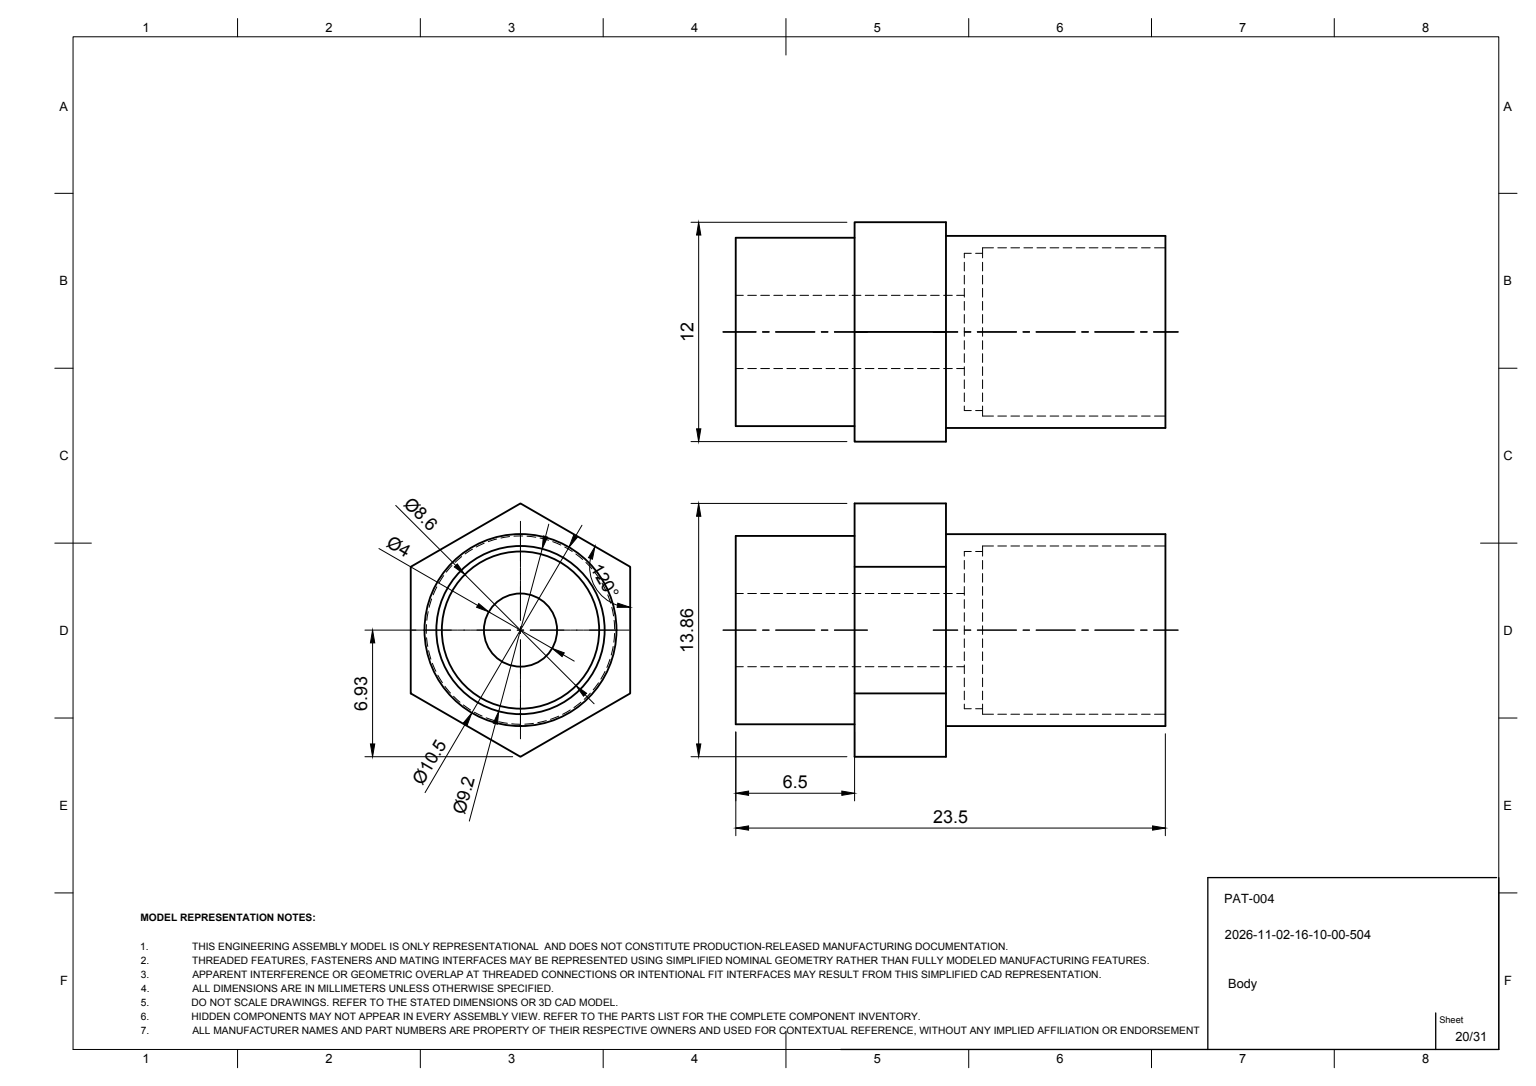
ISO-10303-21;
HEADER;
/* Generated by software containing ST-Developer
 * from STEP Tools, Inc. (www.steptools.com) 
 */

FILE_DESCRIPTION(
/* description */ ('Air blow-off nozzle station'),
/* implementation_level */ '2;1');

FILE_NAME(
/* name */ 'Body.step',
/* time_stamp */ '2026-10-27T10:53:54-07:00',
/* author */ (''),
/* organization */ (''),
/* preprocessor_version */ 'ST-DEVELOPER v20.2',
/* originating_system */ 'Autodesk Translation Framework v15.17.0.0',
/* authorisation */ '');

FILE_SCHEMA (('AUTOMOTIVE_DESIGN { 1 0 10303 214 3 1 1 }'));
ENDSEC;

DATA;
#10=MECHANICAL_DESIGN_GEOMETRIC_PRESENTATION_REPRESENTATION('',(#260),#7897);
#210=SHAPE_REPRESENTATION_RELATIONSHIP('SRR','None',#8028,#235);
#235=ADVANCED_BREP_SHAPE_REPRESENTATION('',(#283),#7895);
#260=STYLED_ITEM('',(#8199),#283);
#283=MANIFOLD_SOLID_BREP('Body1',#4311);
#362=FACE_BOUND('',#1108,.T.);
#363=FACE_BOUND('',#1110,.T.);
#364=FACE_BOUND('',#1112,.T.);
#365=FACE_BOUND('',#1120,.T.);
#366=FACE_BOUND('',#1123,.T.);
#367=FACE_BOUND('',#1127,.T.);
#525=PLANE('',#5017);
#526=PLANE('',#5019);
#527=PLANE('',#5021);
#528=PLANE('',#5023);
#529=PLANE('',#5024);
#530=PLANE('',#5025);
#531=PLANE('',#5026);
#532=PLANE('',#5027);
#533=PLANE('',#5028);
#534=PLANE('',#5029);
#535=PLANE('',#5033);
#536=PLANE('',#5038);
#773=FACE_OUTER_BOUND('',#1106,.T.);
#774=FACE_OUTER_BOUND('',#1107,.T.);
#775=FACE_OUTER_BOUND('',#1109,.T.);
#776=FACE_OUTER_BOUND('',#1111,.T.);
#777=FACE_OUTER_BOUND('',#1113,.T.);
#778=FACE_OUTER_BOUND('',#1114,.T.);
#779=FACE_OUTER_BOUND('',#1115,.T.);
#780=FACE_OUTER_BOUND('',#1116,.T.);
#781=FACE_OUTER_BOUND('',#1117,.T.);
#782=FACE_OUTER_BOUND('',#1118,.T.);
#783=FACE_OUTER_BOUND('',#1119,.T.);
#784=FACE_OUTER_BOUND('',#1121,.T.);
#785=FACE_OUTER_BOUND('',#1122,.T.);
#786=FACE_OUTER_BOUND('',#1124,.T.);
#787=FACE_OUTER_BOUND('',#1125,.T.);
#788=FACE_OUTER_BOUND('',#1126,.T.);
#789=FACE_OUTER_BOUND('',#1128,.T.);
#1106=EDGE_LOOP('',(#3875,#3876,#3877,#3878));
#1107=EDGE_LOOP('',(#3879));
#1108=EDGE_LOOP('',(#3880));
#1109=EDGE_LOOP('',(#3881,#3882,#3883,#3884,#3885,#3886));
#1110=EDGE_LOOP('',(#3887));
#1111=EDGE_LOOP('',(#3888,#3889,#3890,#3891,#3892,#3893));
#1112=EDGE_LOOP('',(#3894));
#1113=EDGE_LOOP('',(#3895,#3896,#3897,#3898));
#1114=EDGE_LOOP('',(#3899,#3900,#3901,#3902));
#1115=EDGE_LOOP('',(#3903,#3904,#3905,#3906));
#1116=EDGE_LOOP('',(#3907,#3908,#3909,#3910));
#1117=EDGE_LOOP('',(#3911,#3912,#3913,#3914));
#1118=EDGE_LOOP('',(#3915,#3916,#3917,#3918));
#1119=EDGE_LOOP('',(#3919));
#1120=EDGE_LOOP('',(#3920));
#1121=EDGE_LOOP('',(#3921,#3922,#3923,#3924));
#1122=EDGE_LOOP('',(#3925));
#1123=EDGE_LOOP('',(#3926));
#1124=EDGE_LOOP('',(#3927,#3928,#3929,#3930));
#1125=EDGE_LOOP('',(#3931,#3932,#3933,#3934));
#1126=EDGE_LOOP('',(#3935));
#1127=EDGE_LOOP('',(#3936));
#1128=EDGE_LOOP('',(#3937,#3938,#3939,#3940));
#1466=LINE('',#7726,#1820);
#1467=LINE('',#7734,#1821);
#1468=LINE('',#7736,#1822);
#1469=LINE('',#7738,#1823);
#1470=LINE('',#7740,#1824);
#1471=LINE('',#7742,#1825);
#1472=LINE('',#7743,#1826);
#1473=LINE('',#7749,#1827);
#1474=LINE('',#7751,#1828);
#1475=LINE('',#7753,#1829);
#1476=LINE('',#7755,#1830);
#1477=LINE('',#7757,#1831);
#1478=LINE('',#7758,#1832);
#1479=LINE('',#7762,#1833);
#1480=LINE('',#7763,#1834);
#1481=LINE('',#7765,#1835);
#1482=LINE('',#7767,#1836);
#1483=LINE('',#7769,#1837);
#1484=LINE('',#7771,#1838);
#1485=LINE('',#7778,#1839);
#1486=LINE('',#7784,#1840);
#1487=LINE('',#7788,#1841);
#1488=LINE('',#7793,#1842);
#1820=VECTOR('',#6254,0.43);
#1821=VECTOR('',#6263,1.);
#1822=VECTOR('',#6264,1.);
#1823=VECTOR('',#6265,1.);
#1824=VECTOR('',#6266,1.);
#1825=VECTOR('',#6267,1.);
#1826=VECTOR('',#6268,1.);
#1827=VECTOR('',#6273,1.);
#1828=VECTOR('',#6274,1.);
#1829=VECTOR('',#6275,1.);
#1830=VECTOR('',#6276,1.);
#1831=VECTOR('',#6277,1.);
#1832=VECTOR('',#6278,1.);
#1833=VECTOR('',#6283,1.);
#1834=VECTOR('',#6284,1.);
#1835=VECTOR('',#6287,1.);
#1836=VECTOR('',#6290,1.);
#1837=VECTOR('',#6293,1.);
#1838=VECTOR('',#6296,1.);
#1839=VECTOR('',#6305,0.46);
#1840=VECTOR('',#6314,0.525);
#1841=VECTOR('',#6319,0.515);
#1842=VECTOR('',#6326,0.2);
#1991=CIRCLE('',#5015,0.43);
#1992=CIRCLE('',#5016,0.43);
#1993=CIRCLE('',#5018,0.2);
#1994=CIRCLE('',#5020,0.525);
#1995=CIRCLE('',#5022,0.515);
#1996=CIRCLE('',#5030,0.46);
#1997=CIRCLE('',#5032,0.46);
#1998=CIRCLE('',#5034,0.525);
#1999=CIRCLE('',#5037,0.515);
#2000=CIRCLE('',#5039,0.2);
#2338=VERTEX_POINT('',#7723);
#2339=VERTEX_POINT('',#7725);
#2340=VERTEX_POINT('',#7729);
#2341=VERTEX_POINT('',#7732);
#2342=VERTEX_POINT('',#7733);
#2343=VERTEX_POINT('',#7735);
#2344=VERTEX_POINT('',#7737);
#2345=VERTEX_POINT('',#7739);
#2346=VERTEX_POINT('',#7741);
#2347=VERTEX_POINT('',#7744);
#2348=VERTEX_POINT('',#7747);
#2349=VERTEX_POINT('',#7748);
#2350=VERTEX_POINT('',#7750);
#2351=VERTEX_POINT('',#7752);
#2352=VERTEX_POINT('',#7754);
#2353=VERTEX_POINT('',#7756);
#2354=VERTEX_POINT('',#7759);
#2355=VERTEX_POINT('',#7774);
#2356=VERTEX_POINT('',#7777);
#2357=VERTEX_POINT('',#7781);
#2358=VERTEX_POINT('',#7786);
#2359=VERTEX_POINT('',#7790);
#2855=EDGE_CURVE('',#2338,#2338,#1991,.T.);
#2856=EDGE_CURVE('',#2338,#2339,#1466,.T.);
#2857=EDGE_CURVE('',#2339,#2339,#1992,.T.);
#2858=EDGE_CURVE('',#2340,#2340,#1993,.T.);
#2859=EDGE_CURVE('',#2341,#2342,#1467,.T.);
#2860=EDGE_CURVE('',#2342,#2343,#1468,.T.);
#2861=EDGE_CURVE('',#2343,#2344,#1469,.T.);
#2862=EDGE_CURVE('',#2344,#2345,#1470,.T.);
#2863=EDGE_CURVE('',#2345,#2346,#1471,.T.);
#2864=EDGE_CURVE('',#2346,#2341,#1472,.T.);
#2865=EDGE_CURVE('',#2347,#2347,#1994,.T.);
#2866=EDGE_CURVE('',#2348,#2349,#1473,.T.);
#2867=EDGE_CURVE('',#2350,#2348,#1474,.T.);
#2868=EDGE_CURVE('',#2351,#2350,#1475,.T.);
#2869=EDGE_CURVE('',#2352,#2351,#1476,.T.);
#2870=EDGE_CURVE('',#2353,#2352,#1477,.T.);
#2871=EDGE_CURVE('',#2349,#2353,#1478,.T.);
#2872=EDGE_CURVE('',#2354,#2354,#1995,.T.);
#2873=EDGE_CURVE('',#2348,#2341,#1479,.T.);
#2874=EDGE_CURVE('',#2350,#2346,#1480,.T.);
#2875=EDGE_CURVE('',#2351,#2345,#1481,.T.);
#2876=EDGE_CURVE('',#2352,#2344,#1482,.T.);
#2877=EDGE_CURVE('',#2353,#2343,#1483,.T.);
#2878=EDGE_CURVE('',#2349,#2342,#1484,.T.);
#2879=EDGE_CURVE('',#2355,#2355,#1996,.T.);
#2880=EDGE_CURVE('',#2355,#2356,#1485,.T.);
#2881=EDGE_CURVE('',#2356,#2356,#1997,.T.);
#2882=EDGE_CURVE('',#2357,#2357,#1998,.T.);
#2883=EDGE_CURVE('',#2347,#2357,#1486,.T.);
#2884=EDGE_CURVE('',#2358,#2358,#1999,.T.);
#2885=EDGE_CURVE('',#2358,#2354,#1487,.T.);
#2886=EDGE_CURVE('',#2359,#2359,#2000,.T.);
#2887=EDGE_CURVE('',#2359,#2340,#1488,.T.);
#3875=ORIENTED_EDGE('',*,*,#2855,.F.);
#3876=ORIENTED_EDGE('',*,*,#2856,.T.);
#3877=ORIENTED_EDGE('',*,*,#2857,.F.);
#3878=ORIENTED_EDGE('',*,*,#2856,.F.);
#3879=ORIENTED_EDGE('',*,*,#2855,.T.);
#3880=ORIENTED_EDGE('',*,*,#2858,.F.);
#3881=ORIENTED_EDGE('',*,*,#2859,.T.);
#3882=ORIENTED_EDGE('',*,*,#2860,.T.);
#3883=ORIENTED_EDGE('',*,*,#2861,.T.);
#3884=ORIENTED_EDGE('',*,*,#2862,.T.);
#3885=ORIENTED_EDGE('',*,*,#2863,.T.);
#3886=ORIENTED_EDGE('',*,*,#2864,.T.);
#3887=ORIENTED_EDGE('',*,*,#2865,.T.);
#3888=ORIENTED_EDGE('',*,*,#2866,.F.);
#3889=ORIENTED_EDGE('',*,*,#2867,.F.);
#3890=ORIENTED_EDGE('',*,*,#2868,.F.);
#3891=ORIENTED_EDGE('',*,*,#2869,.F.);
#3892=ORIENTED_EDGE('',*,*,#2870,.F.);
#3893=ORIENTED_EDGE('',*,*,#2871,.F.);
#3894=ORIENTED_EDGE('',*,*,#2872,.F.);
#3895=ORIENTED_EDGE('',*,*,#2867,.T.);
#3896=ORIENTED_EDGE('',*,*,#2873,.T.);
#3897=ORIENTED_EDGE('',*,*,#2864,.F.);
#3898=ORIENTED_EDGE('',*,*,#2874,.F.);
#3899=ORIENTED_EDGE('',*,*,#2868,.T.);
#3900=ORIENTED_EDGE('',*,*,#2874,.T.);
#3901=ORIENTED_EDGE('',*,*,#2863,.F.);
#3902=ORIENTED_EDGE('',*,*,#2875,.F.);
#3903=ORIENTED_EDGE('',*,*,#2869,.T.);
#3904=ORIENTED_EDGE('',*,*,#2875,.T.);
#3905=ORIENTED_EDGE('',*,*,#2862,.F.);
#3906=ORIENTED_EDGE('',*,*,#2876,.F.);
#3907=ORIENTED_EDGE('',*,*,#2870,.T.);
#3908=ORIENTED_EDGE('',*,*,#2876,.T.);
#3909=ORIENTED_EDGE('',*,*,#2861,.F.);
#3910=ORIENTED_EDGE('',*,*,#2877,.F.);
#3911=ORIENTED_EDGE('',*,*,#2871,.T.);
#3912=ORIENTED_EDGE('',*,*,#2877,.T.);
#3913=ORIENTED_EDGE('',*,*,#2860,.F.);
#3914=ORIENTED_EDGE('',*,*,#2878,.F.);
#3915=ORIENTED_EDGE('',*,*,#2866,.T.);
#3916=ORIENTED_EDGE('',*,*,#2878,.T.);
#3917=ORIENTED_EDGE('',*,*,#2859,.F.);
#3918=ORIENTED_EDGE('',*,*,#2873,.F.);
#3919=ORIENTED_EDGE('',*,*,#2879,.F.);
#3920=ORIENTED_EDGE('',*,*,#2857,.T.);
#3921=ORIENTED_EDGE('',*,*,#2879,.T.);
#3922=ORIENTED_EDGE('',*,*,#2880,.T.);
#3923=ORIENTED_EDGE('',*,*,#2881,.F.);
#3924=ORIENTED_EDGE('',*,*,#2880,.F.);
#3925=ORIENTED_EDGE('',*,*,#2882,.F.);
#3926=ORIENTED_EDGE('',*,*,#2881,.T.);
#3927=ORIENTED_EDGE('',*,*,#2865,.F.);
#3928=ORIENTED_EDGE('',*,*,#2883,.T.);
#3929=ORIENTED_EDGE('',*,*,#2882,.T.);
#3930=ORIENTED_EDGE('',*,*,#2883,.F.);
#3931=ORIENTED_EDGE('',*,*,#2884,.F.);
#3932=ORIENTED_EDGE('',*,*,#2885,.T.);
#3933=ORIENTED_EDGE('',*,*,#2872,.T.);
#3934=ORIENTED_EDGE('',*,*,#2885,.F.);
#3935=ORIENTED_EDGE('',*,*,#2884,.T.);
#3936=ORIENTED_EDGE('',*,*,#2886,.F.);
#3937=ORIENTED_EDGE('',*,*,#2886,.T.);
#3938=ORIENTED_EDGE('',*,*,#2887,.T.);
#3939=ORIENTED_EDGE('',*,*,#2858,.T.);
#3940=ORIENTED_EDGE('',*,*,#2887,.F.);
#4022=CYLINDRICAL_SURFACE('',#5014,0.43);
#4023=CYLINDRICAL_SURFACE('',#5031,0.46);
#4024=CYLINDRICAL_SURFACE('',#5035,0.525);
#4025=CYLINDRICAL_SURFACE('',#5036,0.515);
#4026=CYLINDRICAL_SURFACE('',#5040,0.2);
#4263=ADVANCED_FACE('',(#773),#4022,.F.);
#4264=ADVANCED_FACE('',(#774,#362),#525,.T.);
#4265=ADVANCED_FACE('',(#775,#363),#526,.T.);
#4266=ADVANCED_FACE('',(#776,#364),#527,.F.);
#4267=ADVANCED_FACE('',(#777),#528,.T.);
#4268=ADVANCED_FACE('',(#778),#529,.T.);
#4269=ADVANCED_FACE('',(#779),#530,.T.);
#4270=ADVANCED_FACE('',(#780),#531,.T.);
#4271=ADVANCED_FACE('',(#781),#532,.T.);
#4272=ADVANCED_FACE('',(#782),#533,.T.);
#4273=ADVANCED_FACE('',(#783,#365),#534,.T.);
#4274=ADVANCED_FACE('',(#784),#4023,.F.);
#4275=ADVANCED_FACE('',(#785,#366),#535,.T.);
#4276=ADVANCED_FACE('',(#786),#4024,.T.);
#4277=ADVANCED_FACE('',(#787),#4025,.T.);
#4278=ADVANCED_FACE('',(#788,#367),#536,.T.);
#4279=ADVANCED_FACE('',(#789),#4026,.F.);
#4311=CLOSED_SHELL('',(#4263,#4264,#4265,#4266,#4267,#4268,#4269,#4270,
#4271,#4272,#4273,#4274,#4275,#4276,#4277,#4278,#4279));
#5013=AXIS2_PLACEMENT_3D('',#7721,#6248,#6249);
#5014=AXIS2_PLACEMENT_3D('',#7722,#6250,#6251);
#5015=AXIS2_PLACEMENT_3D('',#7724,#6252,#6253);
#5016=AXIS2_PLACEMENT_3D('',#7727,#6255,#6256);
#5017=AXIS2_PLACEMENT_3D('',#7728,#6257,#6258);
#5018=AXIS2_PLACEMENT_3D('',#7730,#6259,#6260);
#5019=AXIS2_PLACEMENT_3D('',#7731,#6261,#6262);
#5020=AXIS2_PLACEMENT_3D('',#7745,#6269,#6270);
#5021=AXIS2_PLACEMENT_3D('',#7746,#6271,#6272);
#5022=AXIS2_PLACEMENT_3D('',#7760,#6279,#6280);
#5023=AXIS2_PLACEMENT_3D('',#7761,#6281,#6282);
#5024=AXIS2_PLACEMENT_3D('',#7764,#6285,#6286);
#5025=AXIS2_PLACEMENT_3D('',#7766,#6288,#6289);
#5026=AXIS2_PLACEMENT_3D('',#7768,#6291,#6292);
#5027=AXIS2_PLACEMENT_3D('',#7770,#6294,#6295);
#5028=AXIS2_PLACEMENT_3D('',#7772,#6297,#6298);
#5029=AXIS2_PLACEMENT_3D('',#7773,#6299,#6300);
#5030=AXIS2_PLACEMENT_3D('',#7775,#6301,#6302);
#5031=AXIS2_PLACEMENT_3D('',#7776,#6303,#6304);
#5032=AXIS2_PLACEMENT_3D('',#7779,#6306,#6307);
#5033=AXIS2_PLACEMENT_3D('',#7780,#6308,#6309);
#5034=AXIS2_PLACEMENT_3D('',#7782,#6310,#6311);
#5035=AXIS2_PLACEMENT_3D('',#7783,#6312,#6313);
#5036=AXIS2_PLACEMENT_3D('',#7785,#6315,#6316);
#5037=AXIS2_PLACEMENT_3D('',#7787,#6317,#6318);
#5038=AXIS2_PLACEMENT_3D('',#7789,#6320,#6321);
#5039=AXIS2_PLACEMENT_3D('',#7791,#6322,#6323);
#5040=AXIS2_PLACEMENT_3D('',#7792,#6324,#6325);
#6248=DIRECTION('axis',(0.,0.,1.));
#6249=DIRECTION('refdir',(1.,0.,0.));
#6250=DIRECTION('center_axis',(0.,1.,0.));
#6251=DIRECTION('ref_axis',(1.,0.,0.));
#6252=DIRECTION('center_axis',(0.,1.,0.));
#6253=DIRECTION('ref_axis',(1.,0.,0.));
#6254=DIRECTION('',(0.,1.,0.));
#6255=DIRECTION('center_axis',(0.,-1.,0.));
#6256=DIRECTION('ref_axis',(1.,0.,0.));
#6257=DIRECTION('center_axis',(0.,1.,0.));
#6258=DIRECTION('ref_axis',(1.,0.,0.));
#6259=DIRECTION('center_axis',(0.,1.,0.));
#6260=DIRECTION('ref_axis',(1.,0.,0.));
#6261=DIRECTION('center_axis',(0.,1.,0.));
#6262=DIRECTION('ref_axis',(1.,0.,0.));
#6263=DIRECTION('',(0.5,0.,-0.866025403784439));
#6264=DIRECTION('',(-0.5,0.,-0.866025403784439));
#6265=DIRECTION('',(-1.,0.,-1.60246890531964E-16));
#6266=DIRECTION('',(-0.5,0.,0.866025403784439));
#6267=DIRECTION('',(0.5,0.,0.866025403784439));
#6268=DIRECTION('',(1.,0.,1.60246890531964E-16));
#6269=DIRECTION('center_axis',(0.,-1.,0.));
#6270=DIRECTION('ref_axis',(1.,0.,0.));
#6271=DIRECTION('center_axis',(0.,1.,0.));
#6272=DIRECTION('ref_axis',(1.,0.,0.));
#6273=DIRECTION('',(0.5,0.,-0.866025403784439));
#6274=DIRECTION('',(1.,0.,1.60246890531964E-16));
#6275=DIRECTION('',(0.5,0.,0.866025403784439));
#6276=DIRECTION('',(-0.5,0.,0.866025403784439));
#6277=DIRECTION('',(-1.,0.,-1.60246890531964E-16));
#6278=DIRECTION('',(-0.5,0.,-0.866025403784439));
#6279=DIRECTION('center_axis',(0.,-1.,0.));
#6280=DIRECTION('ref_axis',(1.,0.,0.));
#6281=DIRECTION('center_axis',(-1.60246890531964E-16,0.,1.));
#6282=DIRECTION('ref_axis',(1.,0.,1.60246890531964E-16));
#6283=DIRECTION('',(0.,1.,0.));
#6284=DIRECTION('',(0.,1.,0.));
#6285=DIRECTION('center_axis',(-0.866025403784439,0.,0.5));
#6286=DIRECTION('ref_axis',(0.5,0.,0.866025403784439));
#6287=DIRECTION('',(0.,1.,0.));
#6288=DIRECTION('center_axis',(-0.866025403784439,0.,-0.5));
#6289=DIRECTION('ref_axis',(-0.5,0.,0.866025403784439));
#6290=DIRECTION('',(0.,1.,0.));
#6291=DIRECTION('center_axis',(1.60246890531964E-16,0.,-1.));
#6292=DIRECTION('ref_axis',(-1.,0.,-1.60246890531964E-16));
#6293=DIRECTION('',(0.,1.,0.));
#6294=DIRECTION('center_axis',(0.866025403784439,0.,-0.5));
#6295=DIRECTION('ref_axis',(-0.5,0.,-0.866025403784439));
#6296=DIRECTION('',(0.,1.,0.));
#6297=DIRECTION('center_axis',(0.866025403784439,0.,0.5));
#6298=DIRECTION('ref_axis',(0.5,0.,-0.866025403784439));
#6299=DIRECTION('center_axis',(0.,1.,0.));
#6300=DIRECTION('ref_axis',(0.,0.,1.));
#6301=DIRECTION('center_axis',(0.,-1.,0.));
#6302=DIRECTION('ref_axis',(1.,0.,0.));
#6303=DIRECTION('center_axis',(0.,-1.,0.));
#6304=DIRECTION('ref_axis',(1.,0.,0.));
#6305=DIRECTION('',(0.,1.,0.));
#6306=DIRECTION('center_axis',(0.,-1.,0.));
#6307=DIRECTION('ref_axis',(1.,0.,0.));
#6308=DIRECTION('center_axis',(0.,1.,0.));
#6309=DIRECTION('ref_axis',(0.,0.,1.));
#6310=DIRECTION('center_axis',(0.,-1.,0.));
#6311=DIRECTION('ref_axis',(1.,0.,0.));
#6312=DIRECTION('center_axis',(0.,-1.,0.));
#6313=DIRECTION('ref_axis',(1.,0.,0.));
#6314=DIRECTION('',(0.,1.,0.));
#6315=DIRECTION('center_axis',(0.,-1.,0.));
#6316=DIRECTION('ref_axis',(1.,0.,0.));
#6317=DIRECTION('center_axis',(0.,-1.,0.));
#6318=DIRECTION('ref_axis',(1.,0.,0.));
#6319=DIRECTION('',(0.,1.,0.));
#6320=DIRECTION('center_axis',(0.,-1.,0.));
#6321=DIRECTION('ref_axis',(0.,0.,-1.));
#6322=DIRECTION('center_axis',(0.,-1.,0.));
#6323=DIRECTION('ref_axis',(1.,0.,0.));
#6324=DIRECTION('center_axis',(0.,-1.,0.));
#6325=DIRECTION('ref_axis',(1.,0.,0.));
#6326=DIRECTION('',(0.,1.,0.));
#7721=CARTESIAN_POINT('',(0.,0.,0.));
#7722=CARTESIAN_POINT('Origin',(0.,0.6,0.));
#7723=CARTESIAN_POINT('',(-0.43,0.6,5.26598123633362E-17));
#7724=CARTESIAN_POINT('Origin',(0.,0.6,0.));
#7725=CARTESIAN_POINT('',(-0.43,0.7,-5.26598123633362E-17));
#7726=CARTESIAN_POINT('',(-0.43,0.6,5.26598123633362E-17));
#7727=CARTESIAN_POINT('Origin',(0.,0.7,0.));
#7728=CARTESIAN_POINT('Origin',(0.,0.6,0.));
#7729=CARTESIAN_POINT('',(-0.2,0.6,2.44929359829471E-17));
#7730=CARTESIAN_POINT('Origin',(0.,0.6,0.));
#7731=CARTESIAN_POINT('Origin',(0.,0.5,-1.11022302462516E-16));
#7732=CARTESIAN_POINT('',(0.346410161513776,0.5,0.6));
#7733=CARTESIAN_POINT('',(0.692820323027551,0.5,0.));
#7734=CARTESIAN_POINT('',(0.346410161513776,0.5,0.6));
#7735=CARTESIAN_POINT('',(0.346410161513776,0.5,-0.6));
#7736=CARTESIAN_POINT('',(0.692820323027551,0.5,0.));
#7737=CARTESIAN_POINT('',(-0.346410161513775,0.5,-0.6));
#7738=CARTESIAN_POINT('',(0.346410161513776,0.5,-0.6));
#7739=CARTESIAN_POINT('',(-0.692820323027551,0.5,-8.48460190979926E-17));
#7740=CARTESIAN_POINT('',(-0.346410161513775,0.5,-0.6));
#7741=CARTESIAN_POINT('',(-0.346410161513776,0.5,0.6));
#7742=CARTESIAN_POINT('',(-0.692820323027551,0.5,-8.48460190979926E-17));
#7743=CARTESIAN_POINT('',(-0.346410161513776,0.5,0.6));
#7744=CARTESIAN_POINT('',(-0.525,0.5,-6.4293956955236E-17));
#7745=CARTESIAN_POINT('Origin',(0.,0.5,0.));
#7746=CARTESIAN_POINT('Origin',(0.,0.,-1.11022302462516E-16));
#7747=CARTESIAN_POINT('',(0.346410161513776,0.,0.6));
#7748=CARTESIAN_POINT('',(0.692820323027551,0.,0.));
#7749=CARTESIAN_POINT('',(0.346410161513776,0.,0.6));
#7750=CARTESIAN_POINT('',(-0.346410161513776,0.,0.6));
#7751=CARTESIAN_POINT('',(-0.346410161513776,0.,0.6));
#7752=CARTESIAN_POINT('',(-0.692820323027551,0.,-8.48460190979926E-17));
#7753=CARTESIAN_POINT('',(-0.692820323027551,0.,-8.48460190979926E-17));
#7754=CARTESIAN_POINT('',(-0.346410161513775,0.,-0.6));
#7755=CARTESIAN_POINT('',(-0.346410161513775,0.,-0.6));
#7756=CARTESIAN_POINT('',(0.346410161513776,0.,-0.6));
#7757=CARTESIAN_POINT('',(0.346410161513776,0.,-0.6));
#7758=CARTESIAN_POINT('',(0.692820323027551,0.,0.));
#7759=CARTESIAN_POINT('',(-0.515,0.,-6.30693101560887E-17));
#7760=CARTESIAN_POINT('Origin',(0.,0.,0.));
#7761=CARTESIAN_POINT('Origin',(-0.346410161513776,0.,0.6));
#7762=CARTESIAN_POINT('',(0.346410161513776,0.,0.6));
#7763=CARTESIAN_POINT('',(-0.346410161513776,0.,0.6));
#7764=CARTESIAN_POINT('Origin',(-0.692820323027551,0.,-8.48460190979926E-17));
#7765=CARTESIAN_POINT('',(-0.692820323027551,0.,-8.48460190979926E-17));
#7766=CARTESIAN_POINT('Origin',(-0.346410161513775,0.,-0.6));
#7767=CARTESIAN_POINT('',(-0.346410161513775,0.,-0.6));
#7768=CARTESIAN_POINT('Origin',(0.346410161513776,0.,-0.6));
#7769=CARTESIAN_POINT('',(0.346410161513776,0.,-0.6));
#7770=CARTESIAN_POINT('Origin',(0.692820323027551,0.,0.));
#7771=CARTESIAN_POINT('',(0.692820323027551,0.,0.));
#7772=CARTESIAN_POINT('Origin',(0.346410161513776,0.,0.6));
#7773=CARTESIAN_POINT('Origin',(0.46,0.7,0.));
#7774=CARTESIAN_POINT('',(-0.46,0.7,-5.63337527607782E-17));
#7775=CARTESIAN_POINT('Origin',(0.,0.7,0.));
#7776=CARTESIAN_POINT('Origin',(0.,1.2,0.));
#7777=CARTESIAN_POINT('',(-0.46,1.7,-5.63337527607782E-17));
#7778=CARTESIAN_POINT('',(-0.46,1.2,-5.63337527607782E-17));
#7779=CARTESIAN_POINT('Origin',(0.,1.7,0.));
#7780=CARTESIAN_POINT('Origin',(0.525,1.7,0.));
#7781=CARTESIAN_POINT('',(-0.525,1.7,-6.4293956955236E-17));
#7782=CARTESIAN_POINT('Origin',(0.,1.7,0.));
#7783=CARTESIAN_POINT('Origin',(0.,1.1,0.));
#7784=CARTESIAN_POINT('',(-0.525,1.1,-6.4293956955236E-17));
#7785=CARTESIAN_POINT('Origin',(0.,-0.325,0.));
#7786=CARTESIAN_POINT('',(-0.515,-0.65,-6.30693101560887E-17));
#7787=CARTESIAN_POINT('Origin',(0.,-0.65,0.));
#7788=CARTESIAN_POINT('',(-0.515,-0.325,-6.30693101560887E-17));
#7789=CARTESIAN_POINT('Origin',(0.2,-0.65,0.));
#7790=CARTESIAN_POINT('',(-0.2,-0.65,-2.44929359829471E-17));
#7791=CARTESIAN_POINT('Origin',(0.,-0.65,0.));
#7792=CARTESIAN_POINT('Origin',(0.,0.0249999999999999,0.));
#7793=CARTESIAN_POINT('',(-0.2,0.0249999999999999,-2.44929359829471E-17));
#7863=UNCERTAINTY_MEASURE_WITH_UNIT(LENGTH_MEASURE(0.001),#7898,
'DISTANCE_ACCURACY_VALUE',
'Maximum model space distance between geometric entities at asserted c
onnectivities');
#7865=UNCERTAINTY_MEASURE_WITH_UNIT(LENGTH_MEASURE(0.001),#7898,
'DISTANCE_ACCURACY_VALUE',
'Maximum model space distance between geometric entities at asserted c
onnectivities');
#7895=(
GEOMETRIC_REPRESENTATION_CONTEXT(3)
GLOBAL_UNCERTAINTY_ASSIGNED_CONTEXT((#7863))
GLOBAL_UNIT_ASSIGNED_CONTEXT((#7898,#7900,#7901))
REPRESENTATION_CONTEXT('','3D')
);
#7897=(
GEOMETRIC_REPRESENTATION_CONTEXT(3)
GLOBAL_UNCERTAINTY_ASSIGNED_CONTEXT((#7865))
GLOBAL_UNIT_ASSIGNED_CONTEXT((#7898,#7900,#7901))
REPRESENTATION_CONTEXT('','3D')
);
#7898=(
LENGTH_UNIT()
NAMED_UNIT(*)
SI_UNIT(.CENTI.,.METRE.)
);
#7900=(
NAMED_UNIT(*)
PLANE_ANGLE_UNIT()
SI_UNIT($,.RADIAN.)
);
#7901=(
NAMED_UNIT(*)
SI_UNIT($,.STERADIAN.)
SOLID_ANGLE_UNIT()
);
#7931=SHAPE_DEFINITION_REPRESENTATION(#7979,#8028);
#7979=PRODUCT_DEFINITION_SHAPE('',$,#8060);
#8028=SHAPE_REPRESENTATION('',(#5013),#7895);
#8030=PRODUCT_DEFINITION_CONTEXT('part definition',#8125,'design');
#8060=PRODUCT_DEFINITION('Body','Body',#8091,#8030);
#8091=PRODUCT_DEFINITION_FORMATION('',$,#8156);
#8125=APPLICATION_CONTEXT(
'Core Data for Automotive Mechanical Design Process');
#8126=PRODUCT_CONTEXT('part definition',#8125,'mechanical');
#8156=PRODUCT('Body','Body','Body',(#8126));
#8193=COLOUR_RGB('Dark Blue',0.08,0.2,0.34);
#8194=FILL_AREA_STYLE_COLOUR('',#8193);
#8195=FILL_AREA_STYLE('',(#8194));
#8196=SURFACE_STYLE_FILL_AREA(#8195);
#8197=SURFACE_SIDE_STYLE('',(#8196));
#8198=SURFACE_STYLE_USAGE(.BOTH.,#8197);
#8199=PRESENTATION_STYLE_ASSIGNMENT((#8198));
ENDSEC;
END-ISO-10303-21;
